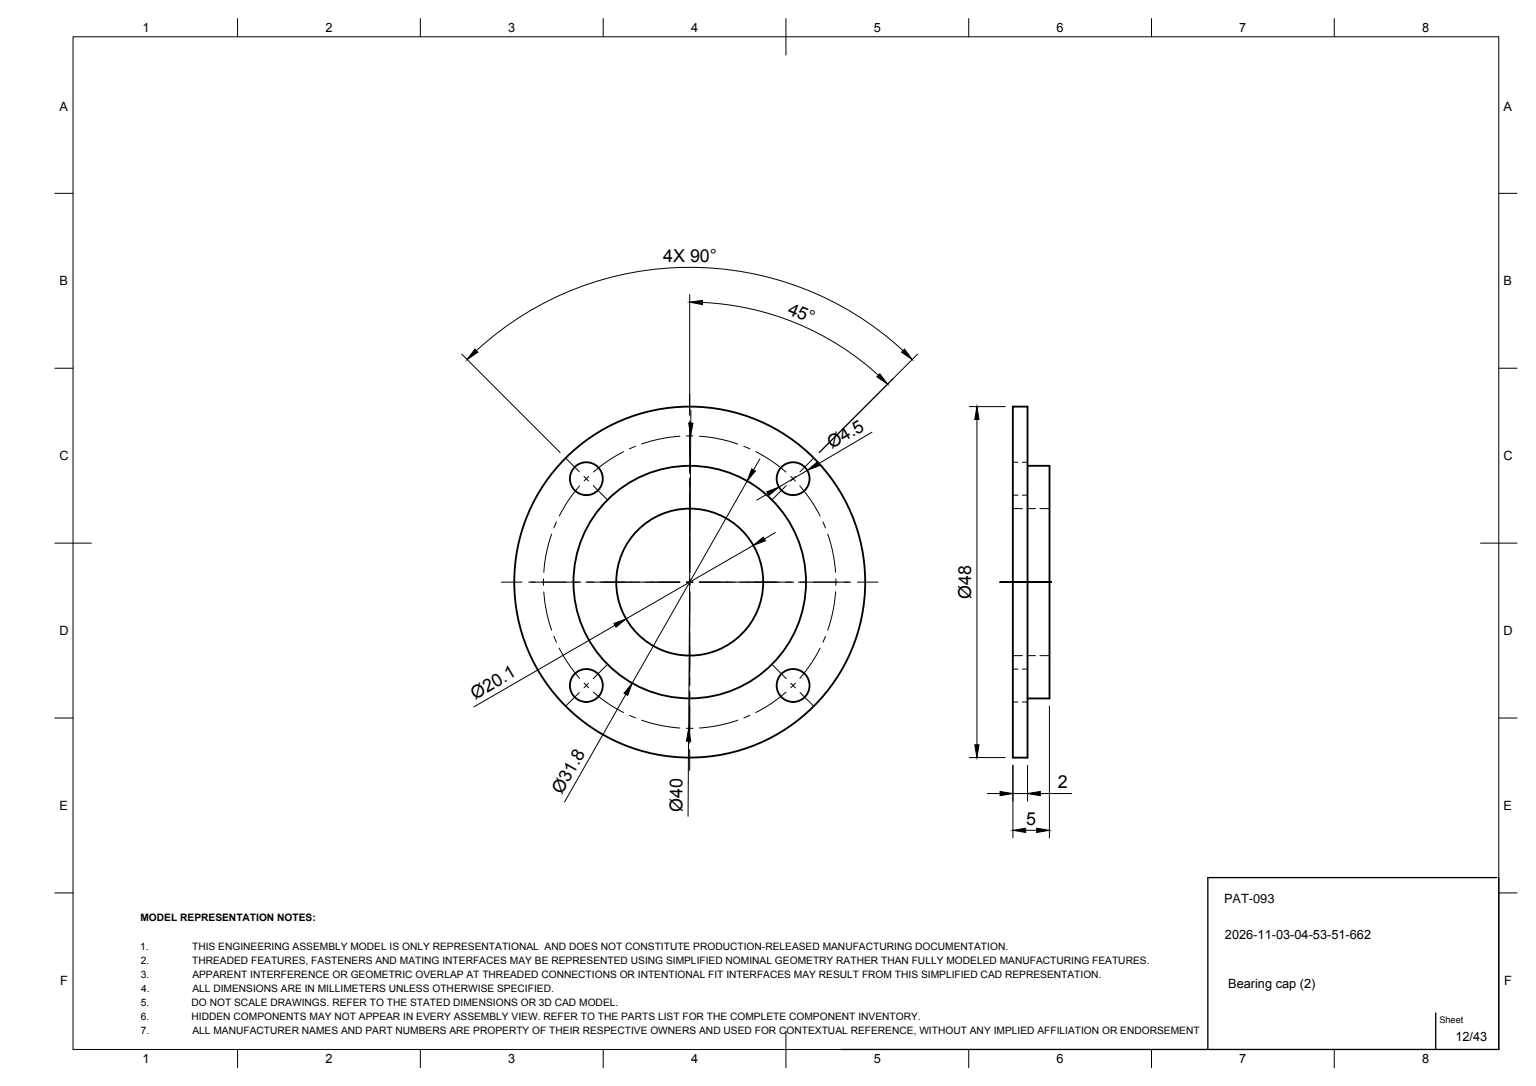
ISO-10303-21;
HEADER;
/* Generated by software containing ST-Developer
 * from STEP Tools, Inc. (www.steptools.com) 
 */

FILE_DESCRIPTION(
/* description */ ('Self-centering screw clamp'),
/* implementation_level */ '2;1');

FILE_NAME(
/* name */ 'Bearing cap (2).step',
/* time_stamp */ '2026-10-28T03:25:31-07:00',
/* author */ (''),
/* organization */ (''),
/* preprocessor_version */ 'ST-DEVELOPER v20.2',
/* originating_system */ 'Autodesk Translation Framework v15.17.0.0',
/* authorisation */ '');

FILE_SCHEMA (('AUTOMOTIVE_DESIGN { 1 0 10303 214 3 1 1 }'));
ENDSEC;

DATA;
#10=MECHANICAL_DESIGN_GEOMETRIC_PRESENTATION_REPRESENTATION('',(#635),#16799);
#553=SHAPE_REPRESENTATION_RELATIONSHIP('SRR','None',#17026,#594);
#594=ADVANCED_BREP_SHAPE_REPRESENTATION('',(#683),#16764);
#635=STYLED_ITEM('',(#17326),#683);
#683=MANIFOLD_SOLID_BREP('Body1',#9086);
#820=FACE_BOUND('',#2041,.T.);
#821=FACE_BOUND('',#2045,.T.);
#822=FACE_BOUND('',#2046,.T.);
#823=FACE_BOUND('',#2047,.T.);
#824=FACE_BOUND('',#2048,.T.);
#825=FACE_BOUND('',#2049,.T.);
#826=FACE_BOUND('',#2051,.T.);
#827=FACE_BOUND('',#2052,.T.);
#828=FACE_BOUND('',#2053,.T.);
#829=FACE_BOUND('',#2054,.T.);
#830=FACE_BOUND('',#2055,.T.);
#1098=PLANE('',#9910);
#1099=PLANE('',#9917);
#1100=PLANE('',#9918);
#1429=FACE_OUTER_BOUND('',#2035,.T.);
#1430=FACE_OUTER_BOUND('',#2036,.T.);
#1431=FACE_OUTER_BOUND('',#2037,.T.);
#1432=FACE_OUTER_BOUND('',#2038,.T.);
#1433=FACE_OUTER_BOUND('',#2039,.T.);
#1434=FACE_OUTER_BOUND('',#2040,.T.);
#1435=FACE_OUTER_BOUND('',#2042,.T.);
#1436=FACE_OUTER_BOUND('',#2043,.T.);
#1437=FACE_OUTER_BOUND('',#2044,.T.);
#1438=FACE_OUTER_BOUND('',#2050,.T.);
#2035=EDGE_LOOP('',(#6895,#6896,#6897,#6898));
#2036=EDGE_LOOP('',(#6899,#6900,#6901,#6902));
#2037=EDGE_LOOP('',(#6903,#6904,#6905,#6906));
#2038=EDGE_LOOP('',(#6907,#6908,#6909,#6910));
#2039=EDGE_LOOP('',(#6911,#6912,#6913,#6914));
#2040=EDGE_LOOP('',(#6915));
#2041=EDGE_LOOP('',(#6916));
#2042=EDGE_LOOP('',(#6917,#6918,#6919,#6920));
#2043=EDGE_LOOP('',(#6921,#6922,#6923,#6924));
#2044=EDGE_LOOP('',(#6925));
#2045=EDGE_LOOP('',(#6926));
#2046=EDGE_LOOP('',(#6927));
#2047=EDGE_LOOP('',(#6928));
#2048=EDGE_LOOP('',(#6929));
#2049=EDGE_LOOP('',(#6930));
#2050=EDGE_LOOP('',(#6931));
#2051=EDGE_LOOP('',(#6932));
#2052=EDGE_LOOP('',(#6933));
#2053=EDGE_LOOP('',(#6934));
#2054=EDGE_LOOP('',(#6935));
#2055=EDGE_LOOP('',(#6936));
#2809=LINE('',#14577,#3382);
#2810=LINE('',#14583,#3383);
#2811=LINE('',#14589,#3384);
#2812=LINE('',#14595,#3385);
#2813=LINE('',#14601,#3386);
#2814=LINE('',#14608,#3387);
#2815=LINE('',#14614,#3388);
#3382=VECTOR('',#11624,0.225);
#3383=VECTOR('',#11631,0.225);
#3384=VECTOR('',#11638,0.225);
#3385=VECTOR('',#11645,0.225);
#3386=VECTOR('',#11652,1.59);
#3387=VECTOR('',#11661,1.005);
#3388=VECTOR('',#11668,2.4);
#3871=CIRCLE('',#9896,0.225);
#3872=CIRCLE('',#9897,0.225);
#3873=CIRCLE('',#9899,0.225);
#3874=CIRCLE('',#9900,0.225);
#3875=CIRCLE('',#9902,0.225);
#3876=CIRCLE('',#9903,0.225);
#3877=CIRCLE('',#9905,0.225);
#3878=CIRCLE('',#9906,0.225);
#3879=CIRCLE('',#9908,1.59);
#3880=CIRCLE('',#9909,1.59);
#3881=CIRCLE('',#9911,1.005);
#3882=CIRCLE('',#9913,1.005);
#3883=CIRCLE('',#9915,2.4);
#3884=CIRCLE('',#9916,2.4);
#4485=VERTEX_POINT('',#14574);
#4486=VERTEX_POINT('',#14576);
#4487=VERTEX_POINT('',#14580);
#4488=VERTEX_POINT('',#14582);
#4489=VERTEX_POINT('',#14586);
#4490=VERTEX_POINT('',#14588);
#4491=VERTEX_POINT('',#14592);
#4492=VERTEX_POINT('',#14594);
#4493=VERTEX_POINT('',#14598);
#4494=VERTEX_POINT('',#14600);
#4495=VERTEX_POINT('',#14604);
#4496=VERTEX_POINT('',#14607);
#4497=VERTEX_POINT('',#14611);
#4498=VERTEX_POINT('',#14613);
#5372=EDGE_CURVE('',#4485,#4485,#3871,.T.);
#5373=EDGE_CURVE('',#4485,#4486,#2809,.T.);
#5374=EDGE_CURVE('',#4486,#4486,#3872,.T.);
#5375=EDGE_CURVE('',#4487,#4487,#3873,.T.);
#5376=EDGE_CURVE('',#4487,#4488,#2810,.T.);
#5377=EDGE_CURVE('',#4488,#4488,#3874,.T.);
#5378=EDGE_CURVE('',#4489,#4489,#3875,.T.);
#5379=EDGE_CURVE('',#4489,#4490,#2811,.T.);
#5380=EDGE_CURVE('',#4490,#4490,#3876,.T.);
#5381=EDGE_CURVE('',#4491,#4491,#3877,.T.);
#5382=EDGE_CURVE('',#4491,#4492,#2812,.T.);
#5383=EDGE_CURVE('',#4492,#4492,#3878,.T.);
#5384=EDGE_CURVE('',#4493,#4493,#3879,.T.);
#5385=EDGE_CURVE('',#4493,#4494,#2813,.T.);
#5386=EDGE_CURVE('',#4494,#4494,#3880,.T.);
#5387=EDGE_CURVE('',#4495,#4495,#3881,.T.);
#5388=EDGE_CURVE('',#4495,#4496,#2814,.T.);
#5389=EDGE_CURVE('',#4496,#4496,#3882,.T.);
#5390=EDGE_CURVE('',#4497,#4497,#3883,.T.);
#5391=EDGE_CURVE('',#4497,#4498,#2815,.T.);
#5392=EDGE_CURVE('',#4498,#4498,#3884,.T.);
#6895=ORIENTED_EDGE('',*,*,#5372,.F.);
#6896=ORIENTED_EDGE('',*,*,#5373,.T.);
#6897=ORIENTED_EDGE('',*,*,#5374,.F.);
#6898=ORIENTED_EDGE('',*,*,#5373,.F.);
#6899=ORIENTED_EDGE('',*,*,#5375,.F.);
#6900=ORIENTED_EDGE('',*,*,#5376,.T.);
#6901=ORIENTED_EDGE('',*,*,#5377,.F.);
#6902=ORIENTED_EDGE('',*,*,#5376,.F.);
#6903=ORIENTED_EDGE('',*,*,#5378,.F.);
#6904=ORIENTED_EDGE('',*,*,#5379,.T.);
#6905=ORIENTED_EDGE('',*,*,#5380,.F.);
#6906=ORIENTED_EDGE('',*,*,#5379,.F.);
#6907=ORIENTED_EDGE('',*,*,#5381,.F.);
#6908=ORIENTED_EDGE('',*,*,#5382,.T.);
#6909=ORIENTED_EDGE('',*,*,#5383,.F.);
#6910=ORIENTED_EDGE('',*,*,#5382,.F.);
#6911=ORIENTED_EDGE('',*,*,#5384,.F.);
#6912=ORIENTED_EDGE('',*,*,#5385,.T.);
#6913=ORIENTED_EDGE('',*,*,#5386,.F.);
#6914=ORIENTED_EDGE('',*,*,#5385,.F.);
#6915=ORIENTED_EDGE('',*,*,#5384,.T.);
#6916=ORIENTED_EDGE('',*,*,#5387,.T.);
#6917=ORIENTED_EDGE('',*,*,#5387,.F.);
#6918=ORIENTED_EDGE('',*,*,#5388,.T.);
#6919=ORIENTED_EDGE('',*,*,#5389,.T.);
#6920=ORIENTED_EDGE('',*,*,#5388,.F.);
#6921=ORIENTED_EDGE('',*,*,#5390,.F.);
#6922=ORIENTED_EDGE('',*,*,#5391,.T.);
#6923=ORIENTED_EDGE('',*,*,#5392,.T.);
#6924=ORIENTED_EDGE('',*,*,#5391,.F.);
#6925=ORIENTED_EDGE('',*,*,#5390,.T.);
#6926=ORIENTED_EDGE('',*,*,#5386,.T.);
#6927=ORIENTED_EDGE('',*,*,#5383,.T.);
#6928=ORIENTED_EDGE('',*,*,#5380,.T.);
#6929=ORIENTED_EDGE('',*,*,#5377,.T.);
#6930=ORIENTED_EDGE('',*,*,#5374,.T.);
#6931=ORIENTED_EDGE('',*,*,#5392,.F.);
#6932=ORIENTED_EDGE('',*,*,#5389,.F.);
#6933=ORIENTED_EDGE('',*,*,#5381,.T.);
#6934=ORIENTED_EDGE('',*,*,#5378,.T.);
#6935=ORIENTED_EDGE('',*,*,#5375,.T.);
#6936=ORIENTED_EDGE('',*,*,#5372,.T.);
#8429=CYLINDRICAL_SURFACE('',#9895,0.225);
#8430=CYLINDRICAL_SURFACE('',#9898,0.225);
#8431=CYLINDRICAL_SURFACE('',#9901,0.225);
#8432=CYLINDRICAL_SURFACE('',#9904,0.225);
#8433=CYLINDRICAL_SURFACE('',#9907,1.59);
#8434=CYLINDRICAL_SURFACE('',#9912,1.005);
#8435=CYLINDRICAL_SURFACE('',#9914,2.4);
#8727=ADVANCED_FACE('',(#1429),#8429,.F.);
#8728=ADVANCED_FACE('',(#1430),#8430,.F.);
#8729=ADVANCED_FACE('',(#1431),#8431,.F.);
#8730=ADVANCED_FACE('',(#1432),#8432,.F.);
#8731=ADVANCED_FACE('',(#1433),#8433,.T.);
#8732=ADVANCED_FACE('',(#1434,#820),#1098,.T.);
#8733=ADVANCED_FACE('',(#1435),#8434,.F.);
#8734=ADVANCED_FACE('',(#1436),#8435,.T.);
#8735=ADVANCED_FACE('',(#1437,#821,#822,#823,#824,#825),#1099,.T.);
#8736=ADVANCED_FACE('',(#1438,#826,#827,#828,#829,#830),#1100,.F.);
#9086=CLOSED_SHELL('',(#8727,#8728,#8729,#8730,#8731,#8732,#8733,#8734,
#8735,#8736));
#9894=AXIS2_PLACEMENT_3D('',#14572,#11618,#11619);
#9895=AXIS2_PLACEMENT_3D('',#14573,#11620,#11621);
#9896=AXIS2_PLACEMENT_3D('',#14575,#11622,#11623);
#9897=AXIS2_PLACEMENT_3D('',#14578,#11625,#11626);
#9898=AXIS2_PLACEMENT_3D('',#14579,#11627,#11628);
#9899=AXIS2_PLACEMENT_3D('',#14581,#11629,#11630);
#9900=AXIS2_PLACEMENT_3D('',#14584,#11632,#11633);
#9901=AXIS2_PLACEMENT_3D('',#14585,#11634,#11635);
#9902=AXIS2_PLACEMENT_3D('',#14587,#11636,#11637);
#9903=AXIS2_PLACEMENT_3D('',#14590,#11639,#11640);
#9904=AXIS2_PLACEMENT_3D('',#14591,#11641,#11642);
#9905=AXIS2_PLACEMENT_3D('',#14593,#11643,#11644);
#9906=AXIS2_PLACEMENT_3D('',#14596,#11646,#11647);
#9907=AXIS2_PLACEMENT_3D('',#14597,#11648,#11649);
#9908=AXIS2_PLACEMENT_3D('',#14599,#11650,#11651);
#9909=AXIS2_PLACEMENT_3D('',#14602,#11653,#11654);
#9910=AXIS2_PLACEMENT_3D('',#14603,#11655,#11656);
#9911=AXIS2_PLACEMENT_3D('',#14605,#11657,#11658);
#9912=AXIS2_PLACEMENT_3D('',#14606,#11659,#11660);
#9913=AXIS2_PLACEMENT_3D('',#14609,#11662,#11663);
#9914=AXIS2_PLACEMENT_3D('',#14610,#11664,#11665);
#9915=AXIS2_PLACEMENT_3D('',#14612,#11666,#11667);
#9916=AXIS2_PLACEMENT_3D('',#14615,#11669,#11670);
#9917=AXIS2_PLACEMENT_3D('',#14616,#11671,#11672);
#9918=AXIS2_PLACEMENT_3D('',#14617,#11673,#11674);
#11618=DIRECTION('axis',(0.,0.,1.));
#11619=DIRECTION('refdir',(1.,0.,0.));
#11620=DIRECTION('center_axis',(1.,0.,0.));
#11621=DIRECTION('ref_axis',(0.,0.,-1.));
#11622=DIRECTION('center_axis',(1.,0.,0.));
#11623=DIRECTION('ref_axis',(0.,0.,-1.));
#11624=DIRECTION('',(1.,0.,0.));
#11625=DIRECTION('center_axis',(-1.,0.,0.));
#11626=DIRECTION('ref_axis',(0.,0.,-1.));
#11627=DIRECTION('center_axis',(1.,0.,0.));
#11628=DIRECTION('ref_axis',(0.,0.,-1.));
#11629=DIRECTION('center_axis',(1.,0.,0.));
#11630=DIRECTION('ref_axis',(0.,0.,-1.));
#11631=DIRECTION('',(1.,0.,0.));
#11632=DIRECTION('center_axis',(-1.,0.,0.));
#11633=DIRECTION('ref_axis',(0.,0.,-1.));
#11634=DIRECTION('center_axis',(1.,0.,0.));
#11635=DIRECTION('ref_axis',(0.,0.,-1.));
#11636=DIRECTION('center_axis',(1.,0.,0.));
#11637=DIRECTION('ref_axis',(0.,0.,-1.));
#11638=DIRECTION('',(1.,0.,0.));
#11639=DIRECTION('center_axis',(-1.,0.,0.));
#11640=DIRECTION('ref_axis',(0.,0.,-1.));
#11641=DIRECTION('center_axis',(1.,0.,0.));
#11642=DIRECTION('ref_axis',(0.,0.,-1.));
#11643=DIRECTION('center_axis',(1.,0.,0.));
#11644=DIRECTION('ref_axis',(0.,0.,-1.));
#11645=DIRECTION('',(1.,0.,0.));
#11646=DIRECTION('center_axis',(-1.,0.,0.));
#11647=DIRECTION('ref_axis',(0.,0.,-1.));
#11648=DIRECTION('center_axis',(1.,0.,0.));
#11649=DIRECTION('ref_axis',(0.,0.,-1.));
#11650=DIRECTION('center_axis',(1.,0.,0.));
#11651=DIRECTION('ref_axis',(0.,0.,-1.));
#11652=DIRECTION('',(-1.,0.,0.));
#11653=DIRECTION('center_axis',(-1.,0.,0.));
#11654=DIRECTION('ref_axis',(0.,0.,-1.));
#11655=DIRECTION('center_axis',(1.,0.,0.));
#11656=DIRECTION('ref_axis',(0.,0.,-1.));
#11657=DIRECTION('center_axis',(-1.,0.,0.));
#11658=DIRECTION('ref_axis',(0.,0.,-1.));
#11659=DIRECTION('center_axis',(1.,0.,0.));
#11660=DIRECTION('ref_axis',(0.,0.,-1.));
#11661=DIRECTION('',(-1.,0.,0.));
#11662=DIRECTION('center_axis',(-1.,0.,0.));
#11663=DIRECTION('ref_axis',(0.,0.,-1.));
#11664=DIRECTION('center_axis',(1.,0.,0.));
#11665=DIRECTION('ref_axis',(0.,0.,-1.));
#11666=DIRECTION('center_axis',(1.,0.,0.));
#11667=DIRECTION('ref_axis',(0.,0.,-1.));
#11668=DIRECTION('',(-1.,0.,0.));
#11669=DIRECTION('center_axis',(1.,0.,0.));
#11670=DIRECTION('ref_axis',(0.,0.,-1.));
#11671=DIRECTION('center_axis',(1.,0.,0.));
#11672=DIRECTION('ref_axis',(0.,0.,-1.));
#11673=DIRECTION('center_axis',(1.,0.,0.));
#11674=DIRECTION('ref_axis',(0.,0.,-1.));
#14572=CARTESIAN_POINT('',(0.,0.,0.));
#14573=CARTESIAN_POINT('Origin',(10.4,-1.4142135623731,2.58578643762691));
#14574=CARTESIAN_POINT('',(10.5,-1.4142135623731,2.81078643762691));
#14575=CARTESIAN_POINT('Origin',(10.5,-1.4142135623731,2.58578643762691));
#14576=CARTESIAN_POINT('',(10.7,-1.4142135623731,2.81078643762691));
#14577=CARTESIAN_POINT('',(10.4,-1.4142135623731,2.81078643762691));
#14578=CARTESIAN_POINT('Origin',(10.7,-1.4142135623731,2.58578643762691));
#14579=CARTESIAN_POINT('Origin',(10.4,-1.41421356237309,5.41421356237309));
#14580=CARTESIAN_POINT('',(10.5,-1.41421356237309,5.63921356237309));
#14581=CARTESIAN_POINT('Origin',(10.5,-1.41421356237309,5.41421356237309));
#14582=CARTESIAN_POINT('',(10.7,-1.41421356237309,5.63921356237309));
#14583=CARTESIAN_POINT('',(10.4,-1.41421356237309,5.63921356237309));
#14584=CARTESIAN_POINT('Origin',(10.7,-1.41421356237309,5.41421356237309));
#14585=CARTESIAN_POINT('Origin',(10.4,1.4142135623731,5.41421356237309));
#14586=CARTESIAN_POINT('',(10.5,1.4142135623731,5.63921356237309));
#14587=CARTESIAN_POINT('Origin',(10.5,1.4142135623731,5.41421356237309));
#14588=CARTESIAN_POINT('',(10.7,1.4142135623731,5.63921356237309));
#14589=CARTESIAN_POINT('',(10.4,1.4142135623731,5.63921356237309));
#14590=CARTESIAN_POINT('Origin',(10.7,1.4142135623731,5.41421356237309));
#14591=CARTESIAN_POINT('Origin',(10.4,1.41421356237309,2.5857864376269));
#14592=CARTESIAN_POINT('',(10.5,1.41421356237309,2.8107864376269));
#14593=CARTESIAN_POINT('Origin',(10.5,1.41421356237309,2.5857864376269));
#14594=CARTESIAN_POINT('',(10.7,1.41421356237309,2.8107864376269));
#14595=CARTESIAN_POINT('',(10.4,1.41421356237309,2.8107864376269));
#14596=CARTESIAN_POINT('Origin',(10.7,1.41421356237309,2.5857864376269));
#14597=CARTESIAN_POINT('Origin',(10.7,0.,4.));
#14598=CARTESIAN_POINT('',(11.,-1.94718841064429E-16,5.59));
#14599=CARTESIAN_POINT('Origin',(11.,0.,4.));
#14600=CARTESIAN_POINT('',(10.7,-1.94718841064429E-16,5.59));
#14601=CARTESIAN_POINT('',(10.7,-1.94718841064429E-16,5.59));
#14602=CARTESIAN_POINT('Origin',(10.7,0.,4.));
#14603=CARTESIAN_POINT('Origin',(11.,0.,4.));
#14604=CARTESIAN_POINT('',(11.,-1.23077003314309E-16,5.005));
#14605=CARTESIAN_POINT('Origin',(11.,0.,4.));
#14606=CARTESIAN_POINT('Origin',(10.5,0.,4.));
#14607=CARTESIAN_POINT('',(10.5,-1.23077003314309E-16,5.005));
#14608=CARTESIAN_POINT('',(10.5,-1.23077003314309E-16,5.005));
#14609=CARTESIAN_POINT('Origin',(10.5,0.,4.));
#14610=CARTESIAN_POINT('Origin',(10.5,0.,4.));
#14611=CARTESIAN_POINT('',(10.7,-2.93915231795365E-16,6.4));
#14612=CARTESIAN_POINT('Origin',(10.7,0.,4.));
#14613=CARTESIAN_POINT('',(10.5,-2.93915231795365E-16,6.4));
#14614=CARTESIAN_POINT('',(10.5,-2.93915231795365E-16,6.4));
#14615=CARTESIAN_POINT('Origin',(10.5,0.,4.));
#14616=CARTESIAN_POINT('Origin',(10.7,0.,4.));
#14617=CARTESIAN_POINT('Origin',(10.5,0.,4.));
#16715=UNCERTAINTY_MEASURE_WITH_UNIT(LENGTH_MEASURE(0.001),#16800,
'DISTANCE_ACCURACY_VALUE',
'Maximum model space distance between geometric entities at asserted c
onnectivities');
#16750=UNCERTAINTY_MEASURE_WITH_UNIT(LENGTH_MEASURE(0.001),#16800,
'DISTANCE_ACCURACY_VALUE',
'Maximum model space distance between geometric entities at asserted c
onnectivities');
#16764=(
GEOMETRIC_REPRESENTATION_CONTEXT(3)
GLOBAL_UNCERTAINTY_ASSIGNED_CONTEXT((#16715))
GLOBAL_UNIT_ASSIGNED_CONTEXT((#16800,#16802,#16803))
REPRESENTATION_CONTEXT('','3D')
);
#16799=(
GEOMETRIC_REPRESENTATION_CONTEXT(3)
GLOBAL_UNCERTAINTY_ASSIGNED_CONTEXT((#16750))
GLOBAL_UNIT_ASSIGNED_CONTEXT((#16800,#16802,#16803))
REPRESENTATION_CONTEXT('','3D')
);
#16800=(
LENGTH_UNIT()
NAMED_UNIT(*)
SI_UNIT(.CENTI.,.METRE.)
);
#16802=(
NAMED_UNIT(*)
PLANE_ANGLE_UNIT()
SI_UNIT($,.RADIAN.)
);
#16803=(
NAMED_UNIT(*)
SI_UNIT($,.STERADIAN.)
SOLID_ANGLE_UNIT()
);
#16817=SHAPE_DEFINITION_REPRESENTATION(#16865,#17026);
#16865=PRODUCT_DEFINITION_SHAPE('',$,#17075);
#17026=SHAPE_REPRESENTATION('',(#9894),#16764);
#17061=PRODUCT_DEFINITION_CONTEXT('part definition',#17207,'design');
#17075=PRODUCT_DEFINITION('Bearing cap (2)','Bearing cap (2)',#17123,#17061);
#17123=PRODUCT_DEFINITION_FORMATION('',$,#17222);
#17207=APPLICATION_CONTEXT(
'Core Data for Automotive Mechanical Design Process');
#17208=PRODUCT_CONTEXT('part definition',#17207,'mechanical');
#17222=PRODUCT('Bearing cap (2)','Bearing cap (2)','Bearing cap (2)',(#17208));
#17320=COLOUR_RGB('Grey',0.48,0.52,0.57);
#17321=FILL_AREA_STYLE_COLOUR('',#17320);
#17322=FILL_AREA_STYLE('',(#17321));
#17323=SURFACE_STYLE_FILL_AREA(#17322);
#17324=SURFACE_SIDE_STYLE('',(#17323));
#17325=SURFACE_STYLE_USAGE(.BOTH.,#17324);
#17326=PRESENTATION_STYLE_ASSIGNMENT((#17325));
ENDSEC;
END-ISO-10303-21;
